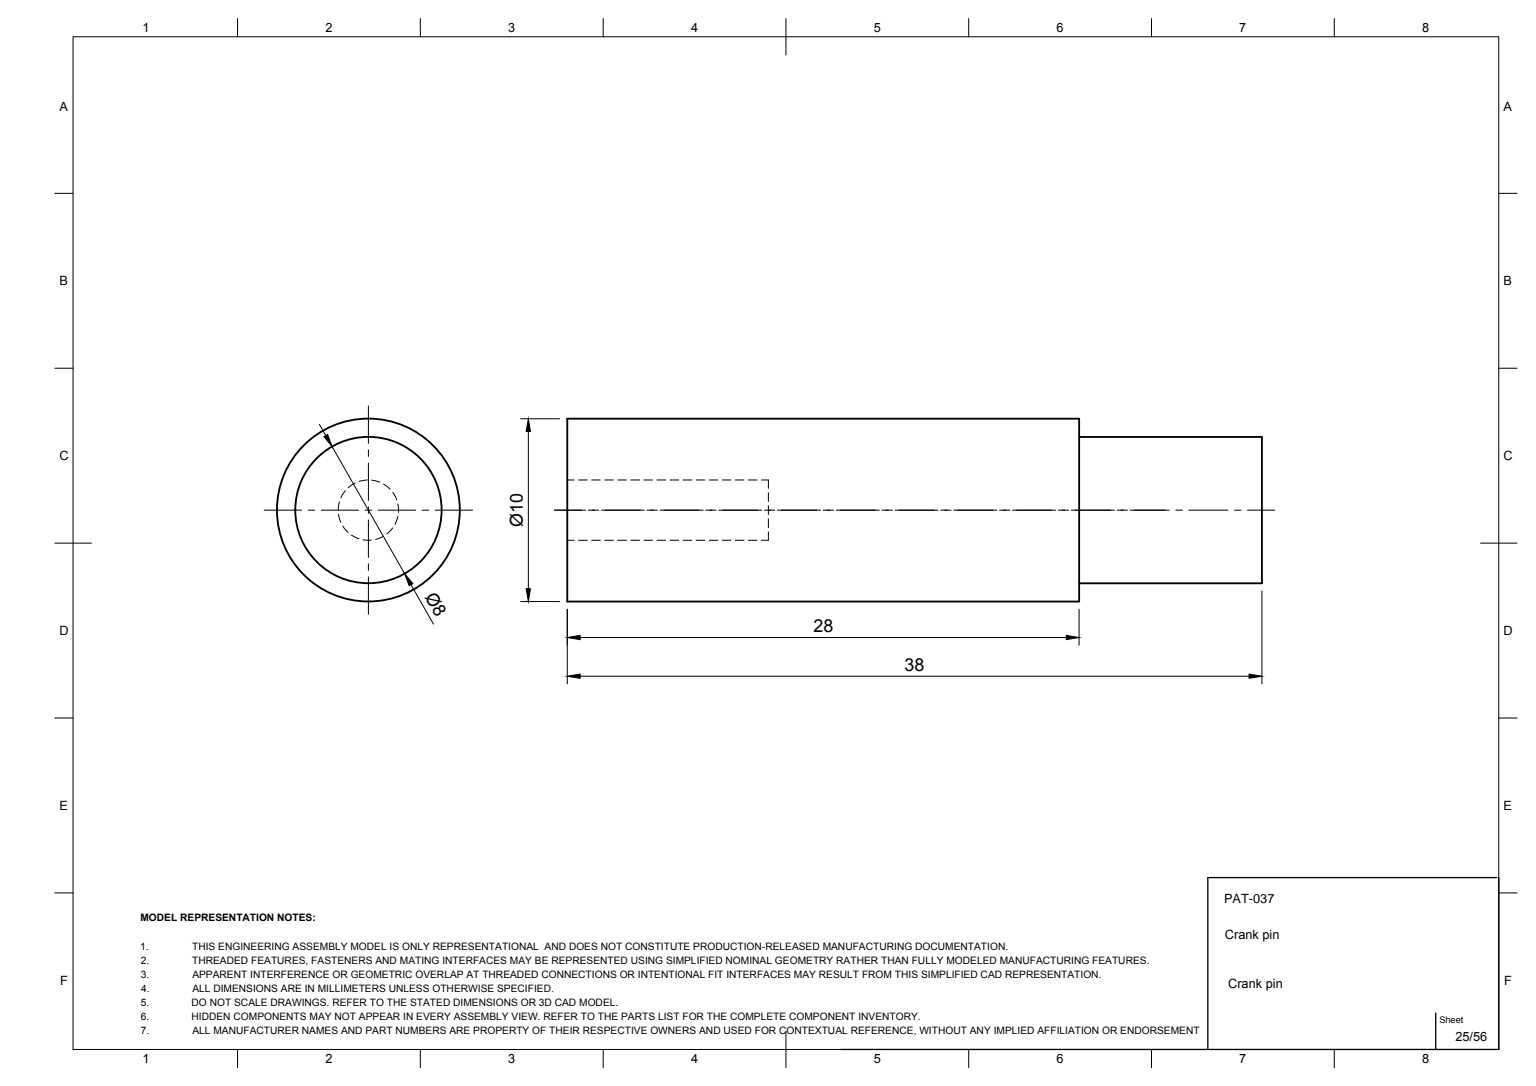
ISO-10303-21;
HEADER;
/* Generated by software containing ST-Developer
 * from STEP Tools, Inc. (www.steptools.com) 
 */

FILE_DESCRIPTION(
/* description */ ('Flywheel Crank-Slider'),
/* implementation_level */ '2;1');

FILE_NAME(
/* name */ 'Crank pin.step',
/* time_stamp */ '2026-10-28T03:23:13-07:00',
/* author */ (''),
/* organization */ (''),
/* preprocessor_version */ 'ST-DEVELOPER v20.2',
/* originating_system */ 'Autodesk Translation Framework v15.17.0.0',
/* authorisation */ '');

FILE_SCHEMA (('AUTOMOTIVE_DESIGN { 1 0 10303 214 3 1 1 }'));
ENDSEC;

DATA;
#10=MECHANICAL_DESIGN_GEOMETRIC_PRESENTATION_REPRESENTATION('',(#695),#17322);
#590=SHAPE_REPRESENTATION_RELATIONSHIP('SRR','None',#17588,#642);
#642=ADVANCED_BREP_SHAPE_REPRESENTATION('',(#752),#17292);
#695=STYLED_ITEM('',(#17931),#752);
#752=MANIFOLD_SOLID_BREP('Body1',#9077);
#922=FACE_BOUND('',#2312,.T.);
#923=FACE_BOUND('',#2315,.T.);
#1201=PLANE('',#10274);
#1202=PLANE('',#10275);
#1203=PLANE('',#10280);
#1204=PLANE('',#10283);
#1637=FACE_OUTER_BOUND('',#2309,.T.);
#1638=FACE_OUTER_BOUND('',#2310,.T.);
#1639=FACE_OUTER_BOUND('',#2311,.T.);
#1640=FACE_OUTER_BOUND('',#2313,.T.);
#1641=FACE_OUTER_BOUND('',#2314,.T.);
#1642=FACE_OUTER_BOUND('',#2316,.T.);
#1643=FACE_OUTER_BOUND('',#2317,.T.);
#2309=EDGE_LOOP('',(#7462,#7463,#7464,#7465));
#2310=EDGE_LOOP('',(#7466));
#2311=EDGE_LOOP('',(#7467));
#2312=EDGE_LOOP('',(#7468));
#2313=EDGE_LOOP('',(#7469,#7470,#7471,#7472));
#2314=EDGE_LOOP('',(#7473));
#2315=EDGE_LOOP('',(#7474));
#2316=EDGE_LOOP('',(#7475,#7476,#7477,#7478));
#2317=EDGE_LOOP('',(#7479));
#3014=LINE('',#15780,#3625);
#3015=LINE('',#15791,#3626);
#3016=LINE('',#15795,#3627);
#3625=VECTOR('',#12404,0.165);
#3626=VECTOR('',#12419,0.5);
#3627=VECTOR('',#12424,0.4);
#4074=CIRCLE('',#10272,0.165);
#4075=CIRCLE('',#10273,0.165);
#4076=CIRCLE('',#10276,0.5);
#4077=CIRCLE('',#10277,0.4);
#4078=CIRCLE('',#10279,0.5);
#4079=CIRCLE('',#10282,0.4);
#4721=VERTEX_POINT('',#15777);
#4722=VERTEX_POINT('',#15779);
#4723=VERTEX_POINT('',#15784);
#4724=VERTEX_POINT('',#15786);
#4725=VERTEX_POINT('',#15789);
#4726=VERTEX_POINT('',#15794);
#5688=EDGE_CURVE('',#4721,#4721,#4074,.T.);
#5689=EDGE_CURVE('',#4721,#4722,#3014,.T.);
#5690=EDGE_CURVE('',#4722,#4722,#4075,.T.);
#5691=EDGE_CURVE('',#4723,#4723,#4076,.T.);
#5692=EDGE_CURVE('',#4724,#4724,#4077,.T.);
#5693=EDGE_CURVE('',#4725,#4725,#4078,.T.);
#5694=EDGE_CURVE('',#4725,#4723,#3015,.T.);
#5695=EDGE_CURVE('',#4724,#4726,#3016,.T.);
#5696=EDGE_CURVE('',#4726,#4726,#4079,.T.);
#7462=ORIENTED_EDGE('',*,*,#5688,.F.);
#7463=ORIENTED_EDGE('',*,*,#5689,.T.);
#7464=ORIENTED_EDGE('',*,*,#5690,.F.);
#7465=ORIENTED_EDGE('',*,*,#5689,.F.);
#7466=ORIENTED_EDGE('',*,*,#5688,.T.);
#7467=ORIENTED_EDGE('',*,*,#5691,.F.);
#7468=ORIENTED_EDGE('',*,*,#5692,.T.);
#7469=ORIENTED_EDGE('',*,*,#5693,.F.);
#7470=ORIENTED_EDGE('',*,*,#5694,.T.);
#7471=ORIENTED_EDGE('',*,*,#5691,.T.);
#7472=ORIENTED_EDGE('',*,*,#5694,.F.);
#7473=ORIENTED_EDGE('',*,*,#5693,.T.);
#7474=ORIENTED_EDGE('',*,*,#5690,.T.);
#7475=ORIENTED_EDGE('',*,*,#5692,.F.);
#7476=ORIENTED_EDGE('',*,*,#5695,.T.);
#7477=ORIENTED_EDGE('',*,*,#5696,.T.);
#7478=ORIENTED_EDGE('',*,*,#5695,.F.);
#7479=ORIENTED_EDGE('',*,*,#5696,.F.);
#8439=CYLINDRICAL_SURFACE('',#10271,0.165);
#8440=CYLINDRICAL_SURFACE('',#10278,0.5);
#8441=CYLINDRICAL_SURFACE('',#10281,0.4);
#8828=ADVANCED_FACE('',(#1637),#8439,.F.);
#8829=ADVANCED_FACE('',(#1638),#1201,.T.);
#8830=ADVANCED_FACE('',(#1639,#922),#1202,.F.);
#8831=ADVANCED_FACE('',(#1640),#8440,.T.);
#8832=ADVANCED_FACE('',(#1641,#923),#1203,.T.);
#8833=ADVANCED_FACE('',(#1642),#8441,.T.);
#8834=ADVANCED_FACE('',(#1643),#1204,.F.);
#9077=CLOSED_SHELL('',(#8828,#8829,#8830,#8831,#8832,#8833,#8834));
#10270=AXIS2_PLACEMENT_3D('',#15775,#12398,#12399);
#10271=AXIS2_PLACEMENT_3D('',#15776,#12400,#12401);
#10272=AXIS2_PLACEMENT_3D('',#15778,#12402,#12403);
#10273=AXIS2_PLACEMENT_3D('',#15781,#12405,#12406);
#10274=AXIS2_PLACEMENT_3D('',#15782,#12407,#12408);
#10275=AXIS2_PLACEMENT_3D('',#15783,#12409,#12410);
#10276=AXIS2_PLACEMENT_3D('',#15785,#12411,#12412);
#10277=AXIS2_PLACEMENT_3D('',#15787,#12413,#12414);
#10278=AXIS2_PLACEMENT_3D('',#15788,#12415,#12416);
#10279=AXIS2_PLACEMENT_3D('',#15790,#12417,#12418);
#10280=AXIS2_PLACEMENT_3D('',#15792,#12420,#12421);
#10281=AXIS2_PLACEMENT_3D('',#15793,#12422,#12423);
#10282=AXIS2_PLACEMENT_3D('',#15796,#12425,#12426);
#10283=AXIS2_PLACEMENT_3D('',#15797,#12427,#12428);
#12398=DIRECTION('axis',(0.,0.,1.));
#12399=DIRECTION('refdir',(1.,0.,0.));
#12400=DIRECTION('center_axis',(0.,1.,0.));
#12401=DIRECTION('ref_axis',(1.,0.,0.));
#12402=DIRECTION('center_axis',(0.,1.,0.));
#12403=DIRECTION('ref_axis',(1.,0.,0.));
#12404=DIRECTION('',(0.,1.,0.));
#12405=DIRECTION('center_axis',(0.,-1.,0.));
#12406=DIRECTION('ref_axis',(1.,0.,0.));
#12407=DIRECTION('center_axis',(0.,1.,0.));
#12408=DIRECTION('ref_axis',(1.,0.,0.));
#12409=DIRECTION('center_axis',(0.,1.,0.));
#12410=DIRECTION('ref_axis',(1.,0.,0.));
#12411=DIRECTION('center_axis',(0.,1.,0.));
#12412=DIRECTION('ref_axis',(1.,0.,0.));
#12413=DIRECTION('center_axis',(0.,1.,0.));
#12414=DIRECTION('ref_axis',(1.,0.,0.));
#12415=DIRECTION('center_axis',(0.,1.,0.));
#12416=DIRECTION('ref_axis',(1.,0.,0.));
#12417=DIRECTION('center_axis',(0.,1.,0.));
#12418=DIRECTION('ref_axis',(1.,0.,0.));
#12419=DIRECTION('',(0.,-1.,0.));
#12420=DIRECTION('center_axis',(0.,1.,0.));
#12421=DIRECTION('ref_axis',(1.,0.,0.));
#12422=DIRECTION('center_axis',(0.,1.,0.));
#12423=DIRECTION('ref_axis',(1.,0.,0.));
#12424=DIRECTION('',(0.,-1.,0.));
#12425=DIRECTION('center_axis',(0.,1.,0.));
#12426=DIRECTION('ref_axis',(1.,0.,0.));
#12427=DIRECTION('center_axis',(0.,1.,0.));
#12428=DIRECTION('ref_axis',(1.,0.,0.));
#15775=CARTESIAN_POINT('',(0.,0.,0.));
#15776=CARTESIAN_POINT('Origin',(2.,2.7,10.));
#15777=CARTESIAN_POINT('',(1.835,2.7,10.));
#15778=CARTESIAN_POINT('Origin',(2.,2.7,10.));
#15779=CARTESIAN_POINT('',(1.835,3.8,10.));
#15780=CARTESIAN_POINT('',(1.835,2.7,10.));
#15781=CARTESIAN_POINT('Origin',(2.,3.8,10.));
#15782=CARTESIAN_POINT('Origin',(2.,2.7,10.));
#15783=CARTESIAN_POINT('Origin',(2.,1.,10.));
#15784=CARTESIAN_POINT('',(1.5,1.,10.));
#15785=CARTESIAN_POINT('Origin',(2.,1.,10.));
#15786=CARTESIAN_POINT('',(1.6,1.,10.));
#15787=CARTESIAN_POINT('Origin',(2.,1.,10.));
#15788=CARTESIAN_POINT('Origin',(2.,1.,10.));
#15789=CARTESIAN_POINT('',(1.5,3.8,10.));
#15790=CARTESIAN_POINT('Origin',(2.,3.8,10.));
#15791=CARTESIAN_POINT('',(1.5,1.,10.));
#15792=CARTESIAN_POINT('Origin',(2.,3.8,10.));
#15793=CARTESIAN_POINT('Origin',(2.,0.,10.));
#15794=CARTESIAN_POINT('',(1.6,0.,10.));
#15795=CARTESIAN_POINT('',(1.6,0.,10.));
#15796=CARTESIAN_POINT('Origin',(2.,0.,10.));
#15797=CARTESIAN_POINT('Origin',(2.,0.,10.));
#17231=UNCERTAINTY_MEASURE_WITH_UNIT(LENGTH_MEASURE(0.001),#17323,
'DISTANCE_ACCURACY_VALUE',
'Maximum model space distance between geometric entities at asserted c
onnectivities');
#17261=UNCERTAINTY_MEASURE_WITH_UNIT(LENGTH_MEASURE(0.001),#17323,
'DISTANCE_ACCURACY_VALUE',
'Maximum model space distance between geometric entities at asserted c
onnectivities');
#17292=(
GEOMETRIC_REPRESENTATION_CONTEXT(3)
GLOBAL_UNCERTAINTY_ASSIGNED_CONTEXT((#17231))
GLOBAL_UNIT_ASSIGNED_CONTEXT((#17323,#17325,#17326))
REPRESENTATION_CONTEXT('','3D')
);
#17322=(
GEOMETRIC_REPRESENTATION_CONTEXT(3)
GLOBAL_UNCERTAINTY_ASSIGNED_CONTEXT((#17261))
GLOBAL_UNIT_ASSIGNED_CONTEXT((#17323,#17325,#17326))
REPRESENTATION_CONTEXT('','3D')
);
#17323=(
LENGTH_UNIT()
NAMED_UNIT(*)
SI_UNIT(.CENTI.,.METRE.)
);
#17325=(
NAMED_UNIT(*)
PLANE_ANGLE_UNIT()
SI_UNIT($,.RADIAN.)
);
#17326=(
NAMED_UNIT(*)
SI_UNIT($,.STERADIAN.)
SOLID_ANGLE_UNIT()
);
#17357=SHAPE_DEFINITION_REPRESENTATION(#17419,#17588);
#17419=PRODUCT_DEFINITION_SHAPE('',$,#17649);
#17588=SHAPE_REPRESENTATION('',(#10270),#17292);
#17618=PRODUCT_DEFINITION_CONTEXT('part definition',#17800,'design');
#17649=PRODUCT_DEFINITION('Crank pin','Crank pin',#17709,#17618);
#17709=PRODUCT_DEFINITION_FORMATION('',$,#17832);
#17800=APPLICATION_CONTEXT(
'Core Data for Automotive Mechanical Design Process');
#17801=PRODUCT_CONTEXT('part definition',#17800,'mechanical');
#17832=PRODUCT('Crank pin','Crank pin','Crank pin',(#17801));
#17925=COLOUR_RGB('Grey',0.48,0.52,0.57);
#17926=FILL_AREA_STYLE_COLOUR('',#17925);
#17927=FILL_AREA_STYLE('',(#17926));
#17928=SURFACE_STYLE_FILL_AREA(#17927);
#17929=SURFACE_SIDE_STYLE('',(#17928));
#17930=SURFACE_STYLE_USAGE(.BOTH.,#17929);
#17931=PRESENTATION_STYLE_ASSIGNMENT((#17930));
ENDSEC;
END-ISO-10303-21;
